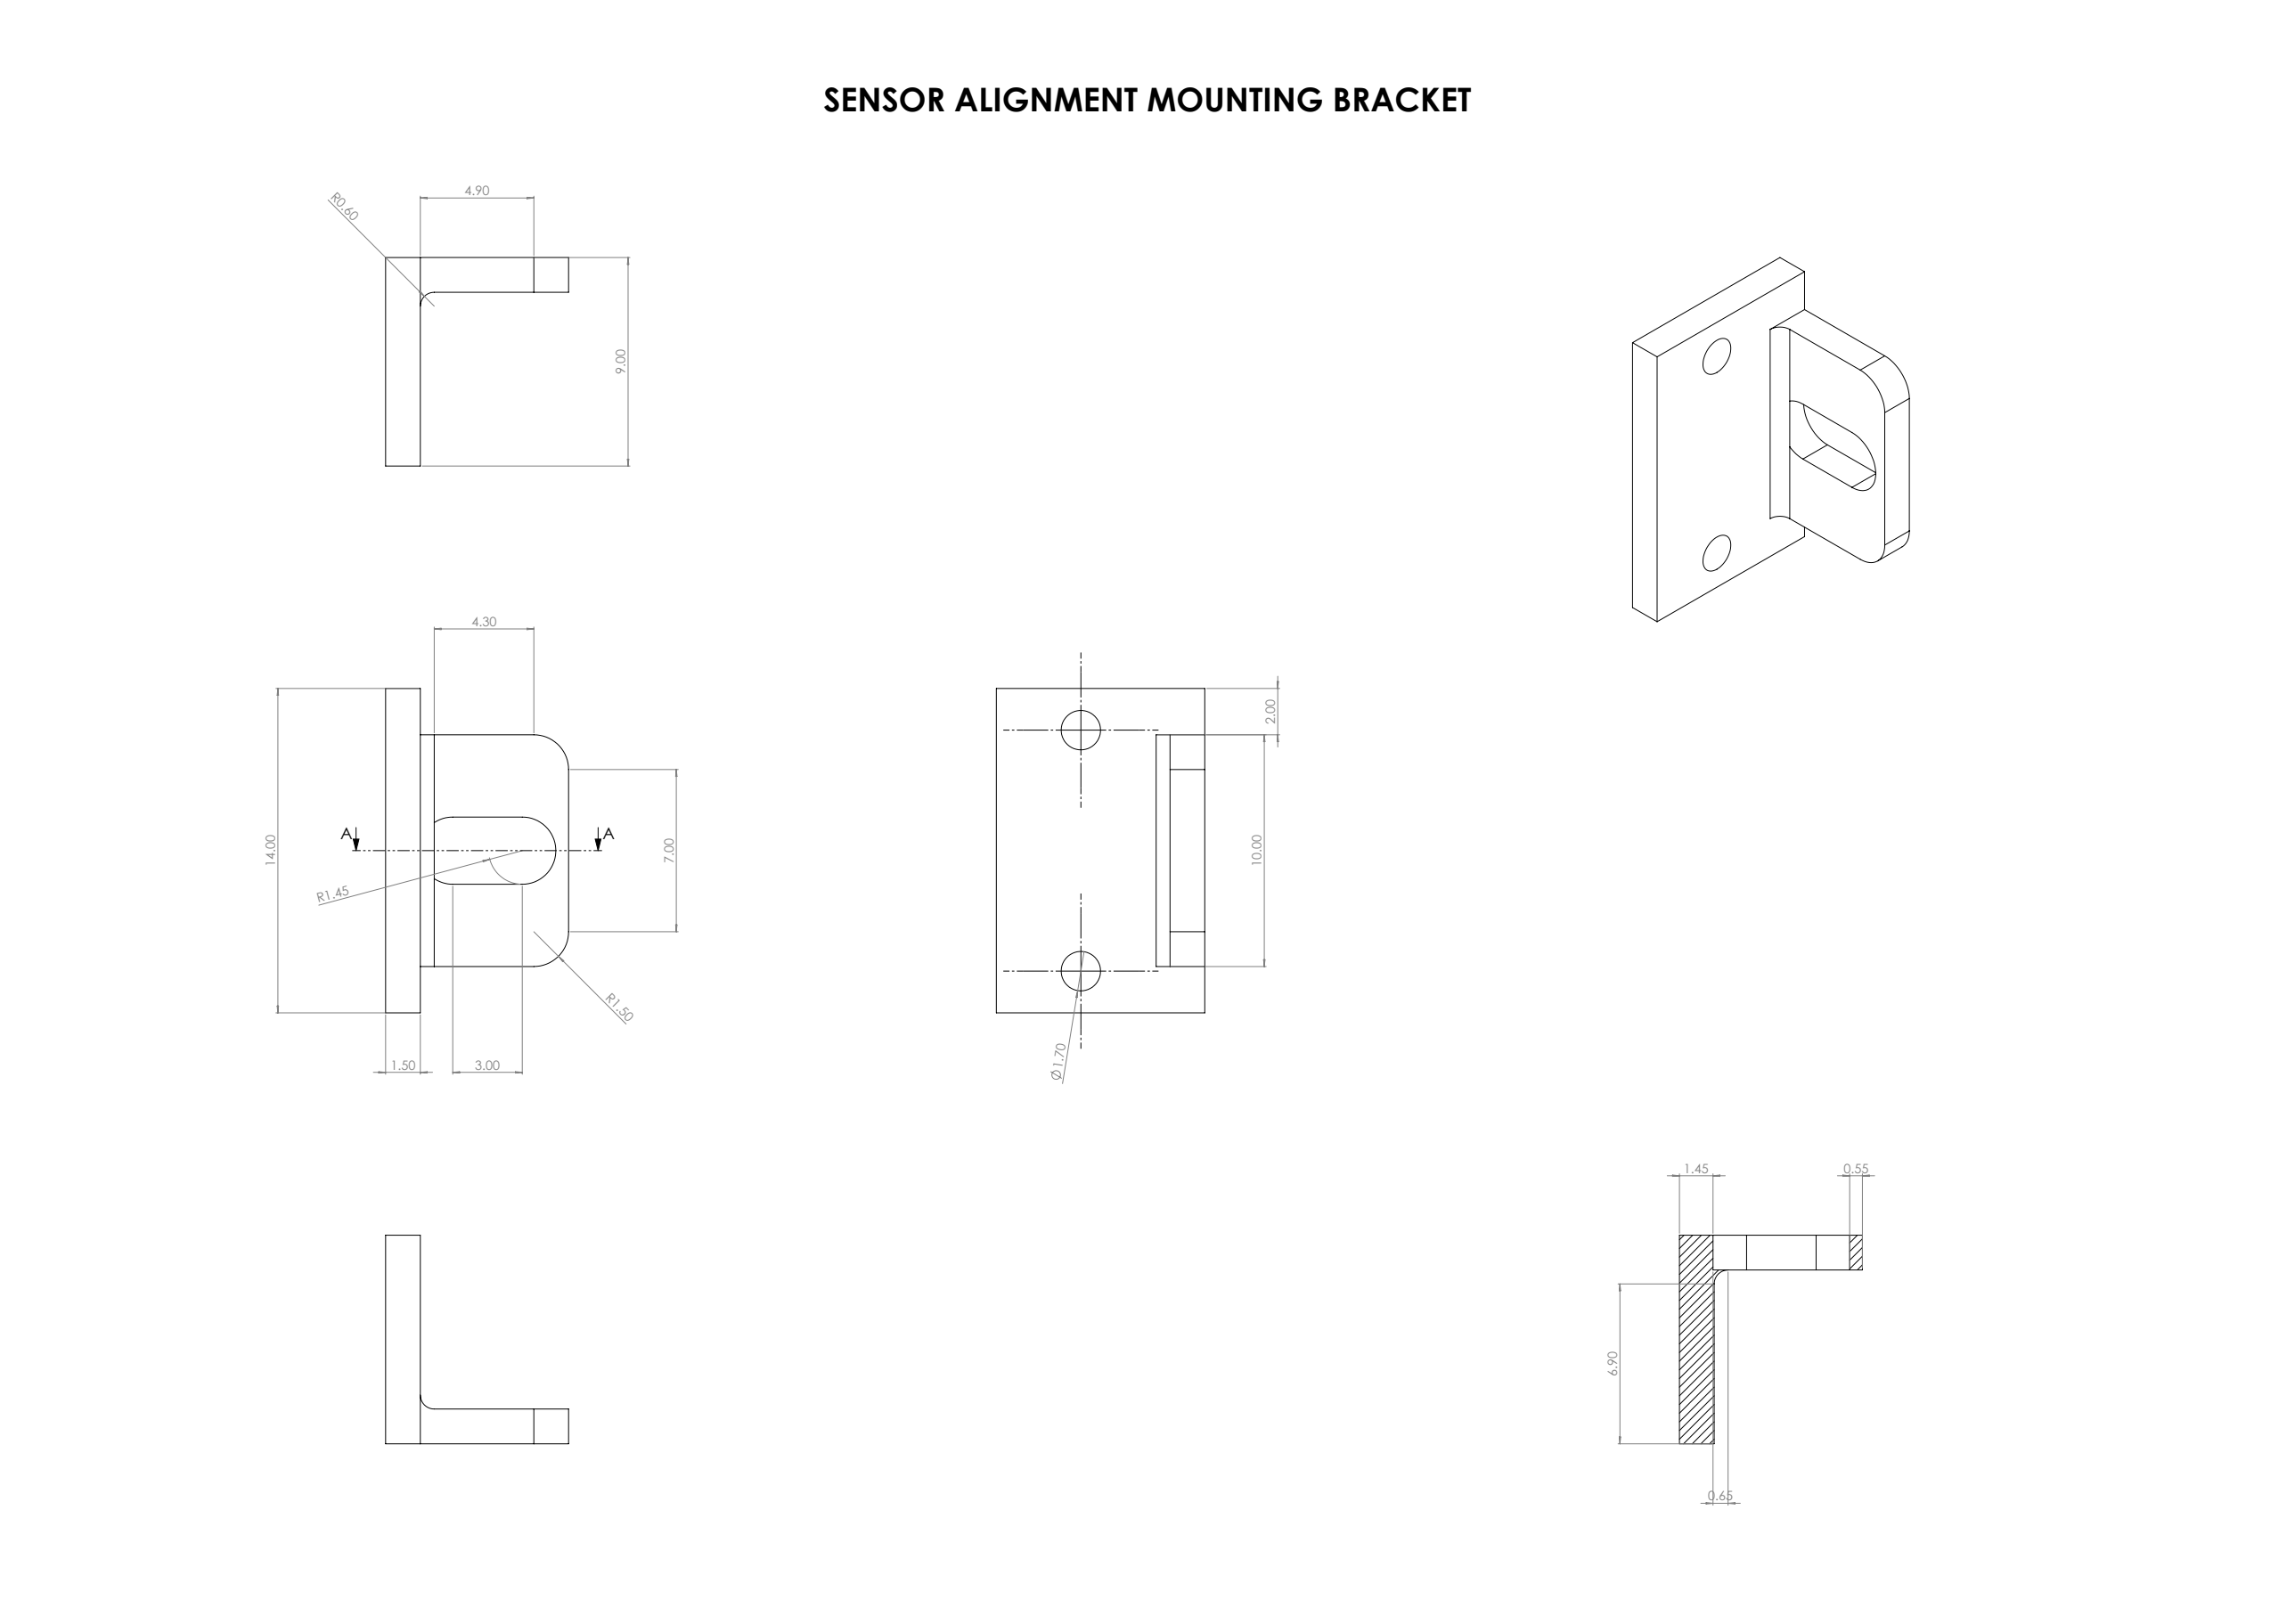
ISO-10303-21;
HEADER;
/* Generated by software containing ST-Developer
 * from STEP Tools, Inc. (www.steptools.com) 
 */

FILE_DESCRIPTION(
/* description */ (''),
/* implementation_level */ '2;1');

FILE_NAME(
/* name */ '12_Sensor_Alignment_Mounting_Bracket.step',
/* time_stamp */ '2026-10-19T23:00:43-07:00',
/* author */ (''),
/* organization */ (''),
/* preprocessor_version */ 'ST-DEVELOPER v20.2',
/* originating_system */ 'Autodesk Translation Framework v15.15.0.0',
/* authorisation */ '');

FILE_SCHEMA (('AUTOMOTIVE_DESIGN { 1 0 10303 214 3 1 1 }'));
ENDSEC;

DATA;
#10=MECHANICAL_DESIGN_GEOMETRIC_PRESENTATION_REPRESENTATION('',(#1007),#55002);
#967=SHAPE_REPRESENTATION_RELATIONSHIP('SRR','None',#55115,#987);
#987=ADVANCED_BREP_SHAPE_REPRESENTATION('',(#1027),#54993);
#1007=STYLED_ITEM('',(#55365),#1027);
#1027=MANIFOLD_SOLID_BREP('Sensor Bracket',#24540);
#1239=FACE_BOUND('',#4618,.T.);
#1240=FACE_BOUND('',#4619,.T.);
#1241=FACE_BOUND('',#4622,.T.);
#1242=FACE_BOUND('',#4623,.T.);
#1243=FACE_BOUND('',#4626,.T.);
#1491=PLANE('',#26066);
#1492=PLANE('',#26071);
#1493=PLANE('',#26080);
#1494=PLANE('',#26083);
#1495=PLANE('',#26087);
#1496=PLANE('',#26091);
#1497=PLANE('',#26092);
#1498=PLANE('',#26093);
#1499=PLANE('',#26094);
#1500=PLANE('',#26095);
#1501=PLANE('',#26096);
#1502=PLANE('',#26097);
#1503=PLANE('',#26098);
#2180=CYLINDRICAL_SURFACE('',#26063,0.15);
#2181=CYLINDRICAL_SURFACE('',#26072,0.15);
#2182=CYLINDRICAL_SURFACE('',#26074,0.085);
#2183=CYLINDRICAL_SURFACE('',#26077,0.085);
#2184=CYLINDRICAL_SURFACE('',#26081,0.145);
#2185=CYLINDRICAL_SURFACE('',#26084,0.145);
#2186=CYLINDRICAL_SURFACE('',#26088,0.06);
#3035=FACE_OUTER_BOUND('',#4602,.T.);
#3036=FACE_OUTER_BOUND('',#4603,.T.);
#3037=FACE_OUTER_BOUND('',#4604,.T.);
#3038=FACE_OUTER_BOUND('',#4605,.T.);
#3039=FACE_OUTER_BOUND('',#4606,.T.);
#3040=FACE_OUTER_BOUND('',#4607,.T.);
#3041=FACE_OUTER_BOUND('',#4608,.T.);
#3042=FACE_OUTER_BOUND('',#4609,.T.);
#3043=FACE_OUTER_BOUND('',#4610,.T.);
#3044=FACE_OUTER_BOUND('',#4611,.T.);
#3045=FACE_OUTER_BOUND('',#4612,.T.);
#3046=FACE_OUTER_BOUND('',#4613,.T.);
#3047=FACE_OUTER_BOUND('',#4614,.T.);
#3048=FACE_OUTER_BOUND('',#4615,.T.);
#3049=FACE_OUTER_BOUND('',#4616,.T.);
#3050=FACE_OUTER_BOUND('',#4617,.T.);
#3051=FACE_OUTER_BOUND('',#4620,.T.);
#3052=FACE_OUTER_BOUND('',#4621,.T.);
#3053=FACE_OUTER_BOUND('',#4624,.T.);
#3054=FACE_OUTER_BOUND('',#4625,.T.);
#4602=EDGE_LOOP('',(#18784,#18785,#18786,#18787));
#4603=EDGE_LOOP('',(#18788,#18789,#18790,#18791,#18792,#18793,#18794,#18795,
#18796,#18797,#18798,#18799));
#4604=EDGE_LOOP('',(#18800,#18801,#18802,#18803));
#4605=EDGE_LOOP('',(#18804,#18805,#18806,#18807));
#4606=EDGE_LOOP('',(#18808,#18809,#18810,#18811));
#4607=EDGE_LOOP('',(#18812,#18813,#18814,#18815));
#4608=EDGE_LOOP('',(#18816,#18817,#18818,#18819));
#4609=EDGE_LOOP('',(#18820,#18821,#18822,#18823));
#4610=EDGE_LOOP('',(#18824,#18825,#18826,#18827));
#4611=EDGE_LOOP('',(#18828,#18829,#18830,#18831,#18832,#18833));
#4612=EDGE_LOOP('',(#18834,#18835));
#4613=EDGE_LOOP('',(#18836,#18837,#18838,#18839,#18840,#18841));
#4614=EDGE_LOOP('',(#18842,#18843,#18844,#18845,#18846));
#4615=EDGE_LOOP('',(#18847,#18848,#18849,#18850,#18851));
#4616=EDGE_LOOP('',(#18852,#18853,#18854,#18855));
#4617=EDGE_LOOP('',(#18856,#18857,#18858,#18859,#18860,#18861,#18862,#18863));
#4618=EDGE_LOOP('',(#18864));
#4619=EDGE_LOOP('',(#18865));
#4620=EDGE_LOOP('',(#18866,#18867,#18868,#18869));
#4621=EDGE_LOOP('',(#18870,#18871,#18872,#18873));
#4622=EDGE_LOOP('',(#18874));
#4623=EDGE_LOOP('',(#18875));
#4624=EDGE_LOOP('',(#18876,#18877,#18878,#18879));
#4625=EDGE_LOOP('',(#18880,#18881,#18882,#18883,#18884,#18885,#18886,#18887,
#18888,#18889));
#4626=EDGE_LOOP('',(#18890,#18891,#18892,#18893));
#6148=LINE('',#37452,#7969);
#6149=LINE('',#37455,#7970);
#6150=LINE('',#37458,#7971);
#6151=LINE('',#37462,#7972);
#6152=LINE('',#37464,#7973);
#6153=LINE('',#37468,#7974);
#6154=LINE('',#37472,#7975);
#6155=LINE('',#37476,#7976);
#6156=LINE('',#37477,#7977);
#6157=LINE('',#37480,#7978);
#6158=LINE('',#37481,#7979);
#6159=LINE('',#37485,#7980);
#6160=LINE('',#37490,#7981);
#6161=LINE('',#37496,#7982);
#6162=LINE('',#37500,#7983);
#6163=LINE('',#37502,#7984);
#6164=LINE('',#37503,#7985);
#6165=LINE('',#37506,#7986);
#6166=LINE('',#37510,#7987);
#6167=LINE('',#37511,#7988);
#6168=LINE('',#37516,#7989);
#6169=LINE('',#37522,#7990);
#6170=LINE('',#37525,#7991);
#6171=LINE('',#37526,#7992);
#6172=LINE('',#37529,#7993);
#6173=LINE('',#37530,#7994);
#6174=LINE('',#37534,#7995);
#6175=LINE('',#37536,#7996);
#6176=LINE('',#37538,#7997);
#6177=LINE('',#37539,#7998);
#6178=LINE('',#37541,#7999);
#6179=LINE('',#37543,#8000);
#6180=LINE('',#37545,#8001);
#6181=LINE('',#37546,#8002);
#6182=LINE('',#37549,#8003);
#6183=LINE('',#37551,#8004);
#6184=LINE('',#37552,#8005);
#6185=LINE('',#37554,#8006);
#6186=LINE('',#37555,#8007);
#7969=VECTOR('',#30554,1.);
#7970=VECTOR('',#30557,1.);
#7971=VECTOR('',#30560,1.);
#7972=VECTOR('',#30563,1.);
#7973=VECTOR('',#30564,1.);
#7974=VECTOR('',#30567,1.);
#7975=VECTOR('',#30570,1.);
#7976=VECTOR('',#30573,1.);
#7977=VECTOR('',#30574,1.);
#7978=VECTOR('',#30577,1.);
#7979=VECTOR('',#30578,1.);
#7980=VECTOR('',#30583,1.);
#7981=VECTOR('',#30588,0.085);
#7982=VECTOR('',#30595,0.085);
#7983=VECTOR('',#30600,1.);
#7984=VECTOR('',#30601,1.);
#7985=VECTOR('',#30602,1.);
#7986=VECTOR('',#30605,1.);
#7987=VECTOR('',#30610,1.);
#7988=VECTOR('',#30611,1.);
#7989=VECTOR('',#30620,1.);
#7990=VECTOR('',#30627,1.);
#7991=VECTOR('',#30630,1.);
#7992=VECTOR('',#30631,1.);
#7993=VECTOR('',#30634,1.);
#7994=VECTOR('',#30635,1.);
#7995=VECTOR('',#30638,1.);
#7996=VECTOR('',#30639,1.);
#7997=VECTOR('',#30640,1.);
#7998=VECTOR('',#30641,1.);
#7999=VECTOR('',#30644,1.);
#8000=VECTOR('',#30645,1.);
#8001=VECTOR('',#30646,1.);
#8002=VECTOR('',#30647,1.);
#8003=VECTOR('',#30650,1.);
#8004=VECTOR('',#30651,1.);
#8005=VECTOR('',#30652,1.);
#8006=VECTOR('',#30655,1.);
#8007=VECTOR('',#30656,1.);
#9682=CIRCLE('',#26064,0.15);
#9683=CIRCLE('',#26065,0.15);
#9684=CIRCLE('',#26067,0.15);
#9685=CIRCLE('',#26068,0.145);
#9686=CIRCLE('',#26069,0.145);
#9687=CIRCLE('',#26070,0.145);
#9688=CIRCLE('',#26073,0.15);
#9689=CIRCLE('',#26075,0.085);
#9690=CIRCLE('',#26076,0.085);
#9691=CIRCLE('',#26078,0.085);
#9692=CIRCLE('',#26079,0.085);
#9693=CIRCLE('',#26082,0.145);
#9694=CIRCLE('',#26085,0.145);
#9695=CIRCLE('',#26086,0.145);
#9696=CIRCLE('',#26089,0.06);
#9697=CIRCLE('',#26090,0.06);
#10965=VERTEX_POINT('',#37448);
#10966=VERTEX_POINT('',#37449);
#10967=VERTEX_POINT('',#37451);
#10968=VERTEX_POINT('',#37453);
#10969=VERTEX_POINT('',#37457);
#10970=VERTEX_POINT('',#37459);
#10971=VERTEX_POINT('',#37461);
#10972=VERTEX_POINT('',#37463);
#10973=VERTEX_POINT('',#37465);
#10974=VERTEX_POINT('',#37467);
#10975=VERTEX_POINT('',#37469);
#10976=VERTEX_POINT('',#37471);
#10977=VERTEX_POINT('',#37473);
#10978=VERTEX_POINT('',#37475);
#10979=VERTEX_POINT('',#37479);
#10980=VERTEX_POINT('',#37483);
#10981=VERTEX_POINT('',#37487);
#10982=VERTEX_POINT('',#37489);
#10983=VERTEX_POINT('',#37493);
#10984=VERTEX_POINT('',#37495);
#10985=VERTEX_POINT('',#37499);
#10986=VERTEX_POINT('',#37501);
#10987=VERTEX_POINT('',#37505);
#10988=VERTEX_POINT('',#37509);
#10989=VERTEX_POINT('',#37518);
#10990=VERTEX_POINT('',#37520);
#10991=VERTEX_POINT('',#37524);
#10992=VERTEX_POINT('',#37528);
#10993=VERTEX_POINT('',#37532);
#10994=VERTEX_POINT('',#37533);
#10995=VERTEX_POINT('',#37535);
#10996=VERTEX_POINT('',#37537);
#10997=VERTEX_POINT('',#37542);
#10998=VERTEX_POINT('',#37544);
#10999=VERTEX_POINT('',#37548);
#11000=VERTEX_POINT('',#37550);
#13800=EDGE_CURVE('',#10965,#10966,#9682,.T.);
#13801=EDGE_CURVE('',#10966,#10967,#6148,.T.);
#13802=EDGE_CURVE('',#10967,#10968,#9683,.T.);
#13803=EDGE_CURVE('',#10968,#10965,#6149,.T.);
#13804=EDGE_CURVE('',#10965,#10969,#6150,.T.);
#13805=EDGE_CURVE('',#10970,#10969,#9684,.T.);
#13806=EDGE_CURVE('',#10970,#10971,#6151,.T.);
#13807=EDGE_CURVE('',#10972,#10971,#6152,.T.);
#13808=EDGE_CURVE('',#10972,#10973,#9685,.T.);
#13809=EDGE_CURVE('',#10973,#10974,#6153,.T.);
#13810=EDGE_CURVE('',#10974,#10975,#9686,.T.);
#13811=EDGE_CURVE('',#10975,#10976,#6154,.T.);
#13812=EDGE_CURVE('',#10976,#10977,#9687,.T.);
#13813=EDGE_CURVE('',#10978,#10977,#6155,.T.);
#13814=EDGE_CURVE('',#10978,#10966,#6156,.T.);
#13815=EDGE_CURVE('',#10968,#10979,#6157,.T.);
#13816=EDGE_CURVE('',#10969,#10979,#6158,.T.);
#13817=EDGE_CURVE('',#10979,#10980,#9688,.T.);
#13818=EDGE_CURVE('',#10980,#10970,#6159,.T.);
#13819=EDGE_CURVE('',#10981,#10981,#9689,.T.);
#13820=EDGE_CURVE('',#10981,#10982,#6160,.T.);
#13821=EDGE_CURVE('',#10982,#10982,#9690,.T.);
#13822=EDGE_CURVE('',#10983,#10983,#9691,.T.);
#13823=EDGE_CURVE('',#10983,#10984,#6161,.T.);
#13824=EDGE_CURVE('',#10984,#10984,#9692,.T.);
#13825=EDGE_CURVE('',#10975,#10985,#6162,.T.);
#13826=EDGE_CURVE('',#10986,#10985,#6163,.T.);
#13827=EDGE_CURVE('',#10976,#10986,#6164,.T.);
#13828=EDGE_CURVE('',#10974,#10987,#6165,.T.);
#13829=EDGE_CURVE('',#10985,#10987,#9693,.T.);
#13830=EDGE_CURVE('',#10973,#10988,#6166,.T.);
#13831=EDGE_CURVE('',#10987,#10988,#6167,.T.);
#13832=EDGE_CURVE('',#10972,#10977,#9694,.T.);
#13833=EDGE_CURVE('',#10988,#10986,#9695,.T.);
#13834=EDGE_CURVE('',#10977,#10972,#6168,.T.);
#13835=EDGE_CURVE('',#10989,#10978,#9696,.T.);
#13836=EDGE_CURVE('',#10971,#10990,#9697,.T.);
#13837=EDGE_CURVE('',#10990,#10989,#6169,.T.);
#13838=EDGE_CURVE('',#10980,#10991,#6170,.T.);
#13839=EDGE_CURVE('',#10990,#10991,#6171,.T.);
#13840=EDGE_CURVE('',#10992,#10989,#6172,.T.);
#13841=EDGE_CURVE('',#10992,#10967,#6173,.T.);
#13842=EDGE_CURVE('',#10993,#10994,#6174,.T.);
#13843=EDGE_CURVE('',#10994,#10995,#6175,.T.);
#13844=EDGE_CURVE('',#10996,#10995,#6176,.T.);
#13845=EDGE_CURVE('',#10993,#10996,#6177,.T.);
#13846=EDGE_CURVE('',#10991,#10993,#6178,.T.);
#13847=EDGE_CURVE('',#10997,#10996,#6179,.T.);
#13848=EDGE_CURVE('',#10998,#10997,#6180,.T.);
#13849=EDGE_CURVE('',#10998,#10992,#6181,.T.);
#13850=EDGE_CURVE('',#10999,#10998,#6182,.T.);
#13851=EDGE_CURVE('',#11000,#10997,#6183,.T.);
#13852=EDGE_CURVE('',#10999,#11000,#6184,.T.);
#13853=EDGE_CURVE('',#10994,#10999,#6185,.T.);
#13854=EDGE_CURVE('',#10995,#11000,#6186,.T.);
#18784=ORIENTED_EDGE('',*,*,#13800,.T.);
#18785=ORIENTED_EDGE('',*,*,#13801,.T.);
#18786=ORIENTED_EDGE('',*,*,#13802,.T.);
#18787=ORIENTED_EDGE('',*,*,#13803,.T.);
#18788=ORIENTED_EDGE('',*,*,#13800,.F.);
#18789=ORIENTED_EDGE('',*,*,#13804,.T.);
#18790=ORIENTED_EDGE('',*,*,#13805,.F.);
#18791=ORIENTED_EDGE('',*,*,#13806,.T.);
#18792=ORIENTED_EDGE('',*,*,#13807,.F.);
#18793=ORIENTED_EDGE('',*,*,#13808,.T.);
#18794=ORIENTED_EDGE('',*,*,#13809,.T.);
#18795=ORIENTED_EDGE('',*,*,#13810,.T.);
#18796=ORIENTED_EDGE('',*,*,#13811,.T.);
#18797=ORIENTED_EDGE('',*,*,#13812,.T.);
#18798=ORIENTED_EDGE('',*,*,#13813,.F.);
#18799=ORIENTED_EDGE('',*,*,#13814,.T.);
#18800=ORIENTED_EDGE('',*,*,#13803,.F.);
#18801=ORIENTED_EDGE('',*,*,#13815,.T.);
#18802=ORIENTED_EDGE('',*,*,#13816,.F.);
#18803=ORIENTED_EDGE('',*,*,#13804,.F.);
#18804=ORIENTED_EDGE('',*,*,#13805,.T.);
#18805=ORIENTED_EDGE('',*,*,#13816,.T.);
#18806=ORIENTED_EDGE('',*,*,#13817,.T.);
#18807=ORIENTED_EDGE('',*,*,#13818,.T.);
#18808=ORIENTED_EDGE('',*,*,#13819,.F.);
#18809=ORIENTED_EDGE('',*,*,#13820,.T.);
#18810=ORIENTED_EDGE('',*,*,#13821,.F.);
#18811=ORIENTED_EDGE('',*,*,#13820,.F.);
#18812=ORIENTED_EDGE('',*,*,#13822,.F.);
#18813=ORIENTED_EDGE('',*,*,#13823,.T.);
#18814=ORIENTED_EDGE('',*,*,#13824,.F.);
#18815=ORIENTED_EDGE('',*,*,#13823,.F.);
#18816=ORIENTED_EDGE('',*,*,#13811,.F.);
#18817=ORIENTED_EDGE('',*,*,#13825,.T.);
#18818=ORIENTED_EDGE('',*,*,#13826,.F.);
#18819=ORIENTED_EDGE('',*,*,#13827,.F.);
#18820=ORIENTED_EDGE('',*,*,#13810,.F.);
#18821=ORIENTED_EDGE('',*,*,#13828,.T.);
#18822=ORIENTED_EDGE('',*,*,#13829,.F.);
#18823=ORIENTED_EDGE('',*,*,#13825,.F.);
#18824=ORIENTED_EDGE('',*,*,#13809,.F.);
#18825=ORIENTED_EDGE('',*,*,#13830,.T.);
#18826=ORIENTED_EDGE('',*,*,#13831,.F.);
#18827=ORIENTED_EDGE('',*,*,#13828,.F.);
#18828=ORIENTED_EDGE('',*,*,#13808,.F.);
#18829=ORIENTED_EDGE('',*,*,#13832,.T.);
#18830=ORIENTED_EDGE('',*,*,#13812,.F.);
#18831=ORIENTED_EDGE('',*,*,#13827,.T.);
#18832=ORIENTED_EDGE('',*,*,#13833,.F.);
#18833=ORIENTED_EDGE('',*,*,#13830,.F.);
#18834=ORIENTED_EDGE('',*,*,#13834,.F.);
#18835=ORIENTED_EDGE('',*,*,#13832,.F.);
#18836=ORIENTED_EDGE('',*,*,#13835,.T.);
#18837=ORIENTED_EDGE('',*,*,#13813,.T.);
#18838=ORIENTED_EDGE('',*,*,#13834,.T.);
#18839=ORIENTED_EDGE('',*,*,#13807,.T.);
#18840=ORIENTED_EDGE('',*,*,#13836,.T.);
#18841=ORIENTED_EDGE('',*,*,#13837,.T.);
#18842=ORIENTED_EDGE('',*,*,#13818,.F.);
#18843=ORIENTED_EDGE('',*,*,#13838,.T.);
#18844=ORIENTED_EDGE('',*,*,#13839,.F.);
#18845=ORIENTED_EDGE('',*,*,#13836,.F.);
#18846=ORIENTED_EDGE('',*,*,#13806,.F.);
#18847=ORIENTED_EDGE('',*,*,#13801,.F.);
#18848=ORIENTED_EDGE('',*,*,#13814,.F.);
#18849=ORIENTED_EDGE('',*,*,#13835,.F.);
#18850=ORIENTED_EDGE('',*,*,#13840,.F.);
#18851=ORIENTED_EDGE('',*,*,#13841,.T.);
#18852=ORIENTED_EDGE('',*,*,#13842,.T.);
#18853=ORIENTED_EDGE('',*,*,#13843,.T.);
#18854=ORIENTED_EDGE('',*,*,#13844,.F.);
#18855=ORIENTED_EDGE('',*,*,#13845,.F.);
#18856=ORIENTED_EDGE('',*,*,#13839,.T.);
#18857=ORIENTED_EDGE('',*,*,#13846,.T.);
#18858=ORIENTED_EDGE('',*,*,#13845,.T.);
#18859=ORIENTED_EDGE('',*,*,#13847,.F.);
#18860=ORIENTED_EDGE('',*,*,#13848,.F.);
#18861=ORIENTED_EDGE('',*,*,#13849,.T.);
#18862=ORIENTED_EDGE('',*,*,#13840,.T.);
#18863=ORIENTED_EDGE('',*,*,#13837,.F.);
#18864=ORIENTED_EDGE('',*,*,#13819,.T.);
#18865=ORIENTED_EDGE('',*,*,#13822,.T.);
#18866=ORIENTED_EDGE('',*,*,#13850,.T.);
#18867=ORIENTED_EDGE('',*,*,#13848,.T.);
#18868=ORIENTED_EDGE('',*,*,#13851,.F.);
#18869=ORIENTED_EDGE('',*,*,#13852,.F.);
#18870=ORIENTED_EDGE('',*,*,#13853,.T.);
#18871=ORIENTED_EDGE('',*,*,#13852,.T.);
#18872=ORIENTED_EDGE('',*,*,#13854,.F.);
#18873=ORIENTED_EDGE('',*,*,#13843,.F.);
#18874=ORIENTED_EDGE('',*,*,#13821,.T.);
#18875=ORIENTED_EDGE('',*,*,#13824,.T.);
#18876=ORIENTED_EDGE('',*,*,#13854,.T.);
#18877=ORIENTED_EDGE('',*,*,#13851,.T.);
#18878=ORIENTED_EDGE('',*,*,#13847,.T.);
#18879=ORIENTED_EDGE('',*,*,#13844,.T.);
#18880=ORIENTED_EDGE('',*,*,#13802,.F.);
#18881=ORIENTED_EDGE('',*,*,#13841,.F.);
#18882=ORIENTED_EDGE('',*,*,#13849,.F.);
#18883=ORIENTED_EDGE('',*,*,#13850,.F.);
#18884=ORIENTED_EDGE('',*,*,#13853,.F.);
#18885=ORIENTED_EDGE('',*,*,#13842,.F.);
#18886=ORIENTED_EDGE('',*,*,#13846,.F.);
#18887=ORIENTED_EDGE('',*,*,#13838,.F.);
#18888=ORIENTED_EDGE('',*,*,#13817,.F.);
#18889=ORIENTED_EDGE('',*,*,#13815,.F.);
#18890=ORIENTED_EDGE('',*,*,#13826,.T.);
#18891=ORIENTED_EDGE('',*,*,#13829,.T.);
#18892=ORIENTED_EDGE('',*,*,#13831,.T.);
#18893=ORIENTED_EDGE('',*,*,#13833,.T.);
#23788=ADVANCED_FACE('',(#3035),#2180,.T.);
#23789=ADVANCED_FACE('',(#3036),#1491,.T.);
#23790=ADVANCED_FACE('',(#3037),#1492,.T.);
#23791=ADVANCED_FACE('',(#3038),#2181,.T.);
#23792=ADVANCED_FACE('',(#3039),#2182,.F.);
#23793=ADVANCED_FACE('',(#3040),#2183,.F.);
#23794=ADVANCED_FACE('',(#3041),#1493,.F.);
#23795=ADVANCED_FACE('',(#3042),#2184,.F.);
#23796=ADVANCED_FACE('',(#3043),#1494,.F.);
#23797=ADVANCED_FACE('',(#3044),#2185,.F.);
#23798=ADVANCED_FACE('',(#3045),#1495,.F.);
#23799=ADVANCED_FACE('',(#3046),#2186,.F.);
#23800=ADVANCED_FACE('',(#3047),#1496,.T.);
#23801=ADVANCED_FACE('',(#3048),#1497,.T.);
#23802=ADVANCED_FACE('',(#3049),#1498,.T.);
#23803=ADVANCED_FACE('',(#3050,#1239,#1240),#1499,.T.);
#23804=ADVANCED_FACE('',(#3051),#1500,.T.);
#23805=ADVANCED_FACE('',(#3052,#1241,#1242),#1501,.T.);
#23806=ADVANCED_FACE('',(#3053),#1502,.T.);
#23807=ADVANCED_FACE('',(#3054,#1243),#1503,.F.);
#24540=CLOSED_SHELL('',(#23788,#23789,#23790,#23791,#23792,#23793,#23794,
#23795,#23796,#23797,#23798,#23799,#23800,#23801,#23802,#23803,#23804,#23805,
#23806,#23807));
#26062=AXIS2_PLACEMENT_3D('',#37446,#30548,#30549);
#26063=AXIS2_PLACEMENT_3D('',#37447,#30550,#30551);
#26064=AXIS2_PLACEMENT_3D('',#37450,#30552,#30553);
#26065=AXIS2_PLACEMENT_3D('',#37454,#30555,#30556);
#26066=AXIS2_PLACEMENT_3D('',#37456,#30558,#30559);
#26067=AXIS2_PLACEMENT_3D('',#37460,#30561,#30562);
#26068=AXIS2_PLACEMENT_3D('',#37466,#30565,#30566);
#26069=AXIS2_PLACEMENT_3D('',#37470,#30568,#30569);
#26070=AXIS2_PLACEMENT_3D('',#37474,#30571,#30572);
#26071=AXIS2_PLACEMENT_3D('',#37478,#30575,#30576);
#26072=AXIS2_PLACEMENT_3D('',#37482,#30579,#30580);
#26073=AXIS2_PLACEMENT_3D('',#37484,#30581,#30582);
#26074=AXIS2_PLACEMENT_3D('',#37486,#30584,#30585);
#26075=AXIS2_PLACEMENT_3D('',#37488,#30586,#30587);
#26076=AXIS2_PLACEMENT_3D('',#37491,#30589,#30590);
#26077=AXIS2_PLACEMENT_3D('',#37492,#30591,#30592);
#26078=AXIS2_PLACEMENT_3D('',#37494,#30593,#30594);
#26079=AXIS2_PLACEMENT_3D('',#37497,#30596,#30597);
#26080=AXIS2_PLACEMENT_3D('',#37498,#30598,#30599);
#26081=AXIS2_PLACEMENT_3D('',#37504,#30603,#30604);
#26082=AXIS2_PLACEMENT_3D('',#37507,#30606,#30607);
#26083=AXIS2_PLACEMENT_3D('',#37508,#30608,#30609);
#26084=AXIS2_PLACEMENT_3D('',#37512,#30612,#30613);
#26085=AXIS2_PLACEMENT_3D('',#37513,#30614,#30615);
#26086=AXIS2_PLACEMENT_3D('',#37514,#30616,#30617);
#26087=AXIS2_PLACEMENT_3D('',#37515,#30618,#30619);
#26088=AXIS2_PLACEMENT_3D('',#37517,#30621,#30622);
#26089=AXIS2_PLACEMENT_3D('',#37519,#30623,#30624);
#26090=AXIS2_PLACEMENT_3D('',#37521,#30625,#30626);
#26091=AXIS2_PLACEMENT_3D('',#37523,#30628,#30629);
#26092=AXIS2_PLACEMENT_3D('',#37527,#30632,#30633);
#26093=AXIS2_PLACEMENT_3D('',#37531,#30636,#30637);
#26094=AXIS2_PLACEMENT_3D('',#37540,#30642,#30643);
#26095=AXIS2_PLACEMENT_3D('',#37547,#30648,#30649);
#26096=AXIS2_PLACEMENT_3D('',#37553,#30653,#30654);
#26097=AXIS2_PLACEMENT_3D('',#37556,#30657,#30658);
#26098=AXIS2_PLACEMENT_3D('',#37557,#30659,#30660);
#30548=DIRECTION('axis',(0.,0.,1.));
#30549=DIRECTION('refdir',(1.,0.,0.));
#30550=DIRECTION('center_axis',(0.,0.,1.));
#30551=DIRECTION('ref_axis',(0.707106781186546,-0.707106781186549,0.));
#30552=DIRECTION('center_axis',(0.,0.,-1.));
#30553=DIRECTION('ref_axis',(0.707106781186546,-0.707106781186549,0.));
#30554=DIRECTION('',(0.,0.,-1.));
#30555=DIRECTION('center_axis',(0.,0.,1.));
#30556=DIRECTION('ref_axis',(0.707106781186546,-0.707106781186549,0.));
#30557=DIRECTION('',(0.,0.,1.));
#30558=DIRECTION('center_axis',(0.,0.,1.));
#30559=DIRECTION('ref_axis',(1.,0.,0.));
#30560=DIRECTION('',(0.,1.,0.));
#30561=DIRECTION('center_axis',(0.,0.,-1.));
#30562=DIRECTION('ref_axis',(0.707106781186548,0.707106781186547,0.));
#30563=DIRECTION('',(-1.,0.,0.));
#30564=DIRECTION('',(0.,1.,0.));
#30565=DIRECTION('center_axis',(0.,0.,-1.));
#30566=DIRECTION('ref_axis',(0.,1.,0.));
#30567=DIRECTION('',(1.,0.,0.));
#30568=DIRECTION('center_axis',(0.,0.,-1.));
#30569=DIRECTION('ref_axis',(-3.0626842058625E-15,-1.,0.));
#30570=DIRECTION('',(-1.,0.,0.));
#30571=DIRECTION('center_axis',(0.,0.,-1.));
#30572=DIRECTION('ref_axis',(0.,1.,0.));
#30573=DIRECTION('',(0.,1.,0.));
#30574=DIRECTION('',(1.,0.,0.));
#30575=DIRECTION('center_axis',(1.,0.,0.));
#30576=DIRECTION('ref_axis',(0.,1.,0.));
#30577=DIRECTION('',(0.,1.,0.));
#30578=DIRECTION('',(0.,0.,-1.));
#30579=DIRECTION('center_axis',(0.,0.,1.));
#30580=DIRECTION('ref_axis',(0.707106781186548,0.707106781186547,0.));
#30581=DIRECTION('center_axis',(0.,0.,1.));
#30582=DIRECTION('ref_axis',(0.707106781186548,0.707106781186547,0.));
#30583=DIRECTION('',(0.,0.,1.));
#30584=DIRECTION('center_axis',(-1.,0.,0.));
#30585=DIRECTION('ref_axis',(0.,-1.,0.));
#30586=DIRECTION('center_axis',(-1.,0.,0.));
#30587=DIRECTION('ref_axis',(0.,-1.,0.));
#30588=DIRECTION('',(-1.,0.,0.));
#30589=DIRECTION('center_axis',(1.,0.,0.));
#30590=DIRECTION('ref_axis',(0.,-1.,0.));
#30591=DIRECTION('center_axis',(-1.,0.,0.));
#30592=DIRECTION('ref_axis',(0.,-1.,0.));
#30593=DIRECTION('center_axis',(-1.,0.,0.));
#30594=DIRECTION('ref_axis',(0.,-1.,0.));
#30595=DIRECTION('',(-1.,0.,0.));
#30596=DIRECTION('center_axis',(1.,0.,0.));
#30597=DIRECTION('ref_axis',(0.,-1.,0.));
#30598=DIRECTION('center_axis',(0.,-1.,0.));
#30599=DIRECTION('ref_axis',(-1.,0.,0.));
#30600=DIRECTION('',(0.,0.,-1.));
#30601=DIRECTION('',(1.,0.,0.));
#30602=DIRECTION('',(0.,0.,-1.));
#30603=DIRECTION('center_axis',(0.,0.,-1.));
#30604=DIRECTION('ref_axis',(-3.0626842058625E-15,-1.,0.));
#30605=DIRECTION('',(0.,0.,-1.));
#30606=DIRECTION('center_axis',(0.,0.,1.));
#30607=DIRECTION('ref_axis',(-3.0626842058625E-15,-1.,0.));
#30608=DIRECTION('center_axis',(0.,1.,0.));
#30609=DIRECTION('ref_axis',(1.,0.,0.));
#30610=DIRECTION('',(0.,0.,-1.));
#30611=DIRECTION('',(-1.,0.,0.));
#30612=DIRECTION('center_axis',(0.,0.,-1.));
#30613=DIRECTION('ref_axis',(0.,1.,0.));
#30614=DIRECTION('center_axis',(0.,0.,1.));
#30615=DIRECTION('ref_axis',(0.,1.,0.));
#30616=DIRECTION('center_axis',(0.,0.,1.));
#30617=DIRECTION('ref_axis',(0.,1.,0.));
#30618=DIRECTION('center_axis',(0.,0.,1.));
#30619=DIRECTION('ref_axis',(1.,0.,0.));
#30620=DIRECTION('',(0.,1.,0.));
#30621=DIRECTION('center_axis',(0.,1.,0.));
#30622=DIRECTION('ref_axis',(-0.707106781186551,0.,-0.707106781186544));
#30623=DIRECTION('center_axis',(0.,-1.,0.));
#30624=DIRECTION('ref_axis',(-0.707106781186551,0.,-0.707106781186544));
#30625=DIRECTION('center_axis',(0.,1.,0.));
#30626=DIRECTION('ref_axis',(-0.707106781186551,0.,-0.707106781186544));
#30627=DIRECTION('',(0.,-1.,0.));
#30628=DIRECTION('center_axis',(0.,1.,0.));
#30629=DIRECTION('ref_axis',(-1.,0.,0.));
#30630=DIRECTION('',(-1.,0.,0.));
#30631=DIRECTION('',(0.,0.,-1.));
#30632=DIRECTION('center_axis',(0.,-1.,0.));
#30633=DIRECTION('ref_axis',(1.,0.,0.));
#30634=DIRECTION('',(0.,0.,1.));
#30635=DIRECTION('',(1.,0.,0.));
#30636=DIRECTION('center_axis',(0.,1.,0.));
#30637=DIRECTION('ref_axis',(-1.,0.,0.));
#30638=DIRECTION('',(-1.,0.,0.));
#30639=DIRECTION('',(0.,0.,1.));
#30640=DIRECTION('',(-1.,0.,0.));
#30641=DIRECTION('',(0.,0.,1.));
#30642=DIRECTION('center_axis',(1.,0.,0.));
#30643=DIRECTION('ref_axis',(0.,1.,0.));
#30644=DIRECTION('',(0.,1.,0.));
#30645=DIRECTION('',(0.,1.,0.));
#30646=DIRECTION('',(0.,0.,1.));
#30647=DIRECTION('',(0.,1.,0.));
#30648=DIRECTION('center_axis',(0.,-1.,0.));
#30649=DIRECTION('ref_axis',(1.,0.,0.));
#30650=DIRECTION('',(1.,0.,0.));
#30651=DIRECTION('',(1.,0.,0.));
#30652=DIRECTION('',(0.,0.,1.));
#30653=DIRECTION('center_axis',(-1.,0.,0.));
#30654=DIRECTION('ref_axis',(0.,-1.,0.));
#30655=DIRECTION('',(0.,-1.,0.));
#30656=DIRECTION('',(0.,-1.,0.));
#30657=DIRECTION('center_axis',(0.,0.,1.));
#30658=DIRECTION('ref_axis',(1.,0.,0.));
#30659=DIRECTION('center_axis',(0.,0.,1.));
#30660=DIRECTION('ref_axis',(1.,0.,0.));
#37446=CARTESIAN_POINT('',(0.,0.,0.));
#37447=CARTESIAN_POINT('Origin',(3.55,-0.35,-0.535));
#37448=CARTESIAN_POINT('',(3.7,-0.35,-0.385));
#37449=CARTESIAN_POINT('',(3.55,-0.5,-0.385));
#37450=CARTESIAN_POINT('Origin',(3.55,-0.35,-0.385));
#37451=CARTESIAN_POINT('',(3.55,-0.5,-0.535));
#37452=CARTESIAN_POINT('',(3.55,-0.5,-0.535));
#37453=CARTESIAN_POINT('',(3.7,-0.35,-0.535));
#37454=CARTESIAN_POINT('Origin',(3.55,-0.35,-0.535));
#37455=CARTESIAN_POINT('',(3.7,-0.35,-0.535));
#37456=CARTESIAN_POINT('Origin',(3.38,0.,-0.385));
#37457=CARTESIAN_POINT('',(3.7,0.35,-0.385));
#37458=CARTESIAN_POINT('',(3.7,-0.5,-0.385));
#37459=CARTESIAN_POINT('',(3.55,0.5,-0.385));
#37460=CARTESIAN_POINT('Origin',(3.55,0.35,-0.385));
#37461=CARTESIAN_POINT('',(3.12,0.5,-0.385));
#37462=CARTESIAN_POINT('',(3.7,0.5,-0.385));
#37463=CARTESIAN_POINT('',(3.12,0.120933866224478,-0.385));
#37464=CARTESIAN_POINT('',(3.12,-0.35,-0.385));
#37465=CARTESIAN_POINT('',(3.2,0.145,-0.385));
#37466=CARTESIAN_POINT('Origin',(3.2,0.,-0.385));
#37467=CARTESIAN_POINT('',(3.5,0.145,-0.385));
#37468=CARTESIAN_POINT('',(3.29,0.145,-0.385));
#37469=CARTESIAN_POINT('',(3.5,-0.145,-0.385));
#37470=CARTESIAN_POINT('Origin',(3.5,-1.38777878078145E-17,-0.385));
#37471=CARTESIAN_POINT('',(3.2,-0.145,-0.385));
#37472=CARTESIAN_POINT('',(3.44,-0.145,-0.385));
#37473=CARTESIAN_POINT('',(3.12,-0.120933866224478,-0.385));
#37474=CARTESIAN_POINT('Origin',(3.2,0.,-0.385));
#37475=CARTESIAN_POINT('',(3.12,-0.5,-0.385));
#37476=CARTESIAN_POINT('',(3.12,-0.35,-0.385));
#37477=CARTESIAN_POINT('',(3.06,-0.5,-0.385));
#37478=CARTESIAN_POINT('Origin',(3.7,-0.5,-0.535));
#37479=CARTESIAN_POINT('',(3.7,0.35,-0.535));
#37480=CARTESIAN_POINT('',(3.7,-0.5,-0.535));
#37481=CARTESIAN_POINT('',(3.7,0.35,-0.535));
#37482=CARTESIAN_POINT('Origin',(3.55,0.35,-0.535));
#37483=CARTESIAN_POINT('',(3.55,0.5,-0.535));
#37484=CARTESIAN_POINT('Origin',(3.55,0.35,-0.535));
#37485=CARTESIAN_POINT('',(3.55,0.5,-0.535));
#37486=CARTESIAN_POINT('Origin',(2.985,-0.52,0.));
#37487=CARTESIAN_POINT('',(3.06,-0.435,-1.04094977927525E-17));
#37488=CARTESIAN_POINT('Origin',(3.06,-0.52,0.));
#37489=CARTESIAN_POINT('',(2.91,-0.435,1.04094977927525E-17));
#37490=CARTESIAN_POINT('',(2.985,-0.435,-1.04094977927525E-17));
#37491=CARTESIAN_POINT('Origin',(2.91,-0.52,0.));
#37492=CARTESIAN_POINT('Origin',(2.985,0.52,0.));
#37493=CARTESIAN_POINT('',(3.06,0.605,-1.04094977927525E-17));
#37494=CARTESIAN_POINT('Origin',(3.06,0.52,0.));
#37495=CARTESIAN_POINT('',(2.91,0.605,1.04094977927525E-17));
#37496=CARTESIAN_POINT('',(2.985,0.605,-1.04094977927525E-17));
#37497=CARTESIAN_POINT('Origin',(2.91,0.52,0.));
#37498=CARTESIAN_POINT('Origin',(3.5,-0.145,-0.385));
#37499=CARTESIAN_POINT('',(3.5,-0.145,-0.535));
#37500=CARTESIAN_POINT('',(3.5,-0.145,-0.385));
#37501=CARTESIAN_POINT('',(3.2,-0.145,-0.535));
#37502=CARTESIAN_POINT('',(3.2425,-0.145,-0.535));
#37503=CARTESIAN_POINT('',(3.2,-0.145,-0.385));
#37504=CARTESIAN_POINT('Origin',(3.5,-1.38777878078145E-17,-0.385));
#37505=CARTESIAN_POINT('',(3.5,0.145,-0.535));
#37506=CARTESIAN_POINT('',(3.5,0.145,-0.385));
#37507=CARTESIAN_POINT('Origin',(3.5,-1.38777878078145E-17,-0.535));
#37508=CARTESIAN_POINT('Origin',(3.2,0.145,-0.385));
#37509=CARTESIAN_POINT('',(3.2,0.145,-0.535));
#37510=CARTESIAN_POINT('',(3.2,0.145,-0.385));
#37511=CARTESIAN_POINT('',(3.0925,0.145,-0.535));
#37512=CARTESIAN_POINT('Origin',(3.2,0.,-0.385));
#37513=CARTESIAN_POINT('Origin',(3.2,0.,-0.385));
#37514=CARTESIAN_POINT('Origin',(3.2,0.,-0.535));
#37515=CARTESIAN_POINT('Origin',(3.35,0.,-0.385));
#37516=CARTESIAN_POINT('',(3.12,-0.35,-0.385));
#37517=CARTESIAN_POINT('Origin',(3.12,-0.35,-0.325));
#37518=CARTESIAN_POINT('',(3.06,-0.5,-0.325));
#37519=CARTESIAN_POINT('Origin',(3.12,-0.5,-0.325));
#37520=CARTESIAN_POINT('',(3.06,0.5,-0.325));
#37521=CARTESIAN_POINT('Origin',(3.12,0.5,-0.325));
#37522=CARTESIAN_POINT('',(3.06,-0.35,-0.325));
#37523=CARTESIAN_POINT('Origin',(3.7,0.5,-0.535));
#37524=CARTESIAN_POINT('',(3.06,0.5,-0.535));
#37525=CARTESIAN_POINT('',(3.7,0.5,-0.535));
#37526=CARTESIAN_POINT('',(3.06,0.5,-0.535));
#37527=CARTESIAN_POINT('Origin',(3.06,-0.5,-0.535));
#37528=CARTESIAN_POINT('',(3.06,-0.5,-0.535));
#37529=CARTESIAN_POINT('',(3.06,-0.5,-0.535));
#37530=CARTESIAN_POINT('',(3.06,-0.5,-0.535));
#37531=CARTESIAN_POINT('Origin',(3.06,0.7,-0.535));
#37532=CARTESIAN_POINT('',(3.06,0.7,-0.535));
#37533=CARTESIAN_POINT('',(2.91,0.7,-0.535));
#37534=CARTESIAN_POINT('',(3.06,0.7,-0.535));
#37535=CARTESIAN_POINT('',(2.91,0.7,0.365));
#37536=CARTESIAN_POINT('',(2.91,0.7,-0.535));
#37537=CARTESIAN_POINT('',(3.06,0.7,0.365));
#37538=CARTESIAN_POINT('',(3.06,0.7,0.365));
#37539=CARTESIAN_POINT('',(3.06,0.7,-0.535));
#37540=CARTESIAN_POINT('Origin',(3.06,-0.7,-0.535));
#37541=CARTESIAN_POINT('',(3.06,-0.7,-0.535));
#37542=CARTESIAN_POINT('',(3.06,-0.7,0.365));
#37543=CARTESIAN_POINT('',(3.06,-0.7,0.365));
#37544=CARTESIAN_POINT('',(3.06,-0.7,-0.535));
#37545=CARTESIAN_POINT('',(3.06,-0.7,-0.535));
#37546=CARTESIAN_POINT('',(3.06,-0.7,-0.535));
#37547=CARTESIAN_POINT('Origin',(2.91,-0.7,-0.535));
#37548=CARTESIAN_POINT('',(2.91,-0.7,-0.535));
#37549=CARTESIAN_POINT('',(2.91,-0.7,-0.535));
#37550=CARTESIAN_POINT('',(2.91,-0.7,0.365));
#37551=CARTESIAN_POINT('',(2.91,-0.7,0.365));
#37552=CARTESIAN_POINT('',(2.91,-0.7,-0.535));
#37553=CARTESIAN_POINT('Origin',(2.91,0.7,-0.535));
#37554=CARTESIAN_POINT('',(2.91,0.7,-0.535));
#37555=CARTESIAN_POINT('',(2.91,0.7,0.365));
#37556=CARTESIAN_POINT('Origin',(2.985,0.,0.365));
#37557=CARTESIAN_POINT('Origin',(2.985,0.,-0.535));
#54971=UNCERTAINTY_MEASURE_WITH_UNIT(LENGTH_MEASURE(0.001),#55003,
'DISTANCE_ACCURACY_VALUE',
'Maximum model space distance between geometric entities at asserted c
onnectivities');
#54980=UNCERTAINTY_MEASURE_WITH_UNIT(LENGTH_MEASURE(0.001),#55003,
'DISTANCE_ACCURACY_VALUE',
'Maximum model space distance between geometric entities at asserted c
onnectivities');
#54993=(
GEOMETRIC_REPRESENTATION_CONTEXT(3)
GLOBAL_UNCERTAINTY_ASSIGNED_CONTEXT((#54971))
GLOBAL_UNIT_ASSIGNED_CONTEXT((#55003,#55005,#55006))
REPRESENTATION_CONTEXT('','3D')
);
#55002=(
GEOMETRIC_REPRESENTATION_CONTEXT(3)
GLOBAL_UNCERTAINTY_ASSIGNED_CONTEXT((#54980))
GLOBAL_UNIT_ASSIGNED_CONTEXT((#55003,#55005,#55006))
REPRESENTATION_CONTEXT('','3D')
);
#55003=(
LENGTH_UNIT()
NAMED_UNIT(*)
SI_UNIT(.CENTI.,.METRE.)
);
#55005=(
NAMED_UNIT(*)
PLANE_ANGLE_UNIT()
SI_UNIT($,.RADIAN.)
);
#55006=(
NAMED_UNIT(*)
SI_UNIT($,.STERADIAN.)
SOLID_ANGLE_UNIT()
);
#55019=SHAPE_DEFINITION_REPRESENTATION(#55040,#55115);
#55040=PRODUCT_DEFINITION_SHAPE('',$,#55137);
#55115=SHAPE_REPRESENTATION('',(#26062),#54993);
#55124=PRODUCT_DEFINITION_CONTEXT('part definition',#55189,'design');
#55137=PRODUCT_DEFINITION('2026-10-18-23-36-34-140',
'12_Sensor_Alignment_Mounting_Bracket',#55158,#55124);
#55158=PRODUCT_DEFINITION_FORMATION('',$,#55203);
#55189=APPLICATION_CONTEXT(
'Core Data for Automotive Mechanical Design Process');
#55190=PRODUCT_CONTEXT('part definition',#55189,'mechanical');
#55203=PRODUCT('2026-10-18-23-36-34-140',
'12_Sensor_Alignment_Mounting_Bracket',$,(#55190));
#55359=COLOUR_RGB('Dark Blue',0.08,0.2,0.34);
#55360=FILL_AREA_STYLE_COLOUR('',#55359);
#55361=FILL_AREA_STYLE('',(#55360));
#55362=SURFACE_STYLE_FILL_AREA(#55361);
#55363=SURFACE_SIDE_STYLE('',(#55362));
#55364=SURFACE_STYLE_USAGE(.BOTH.,#55363);
#55365=PRESENTATION_STYLE_ASSIGNMENT((#55364));
ENDSEC;
END-ISO-10303-21;
